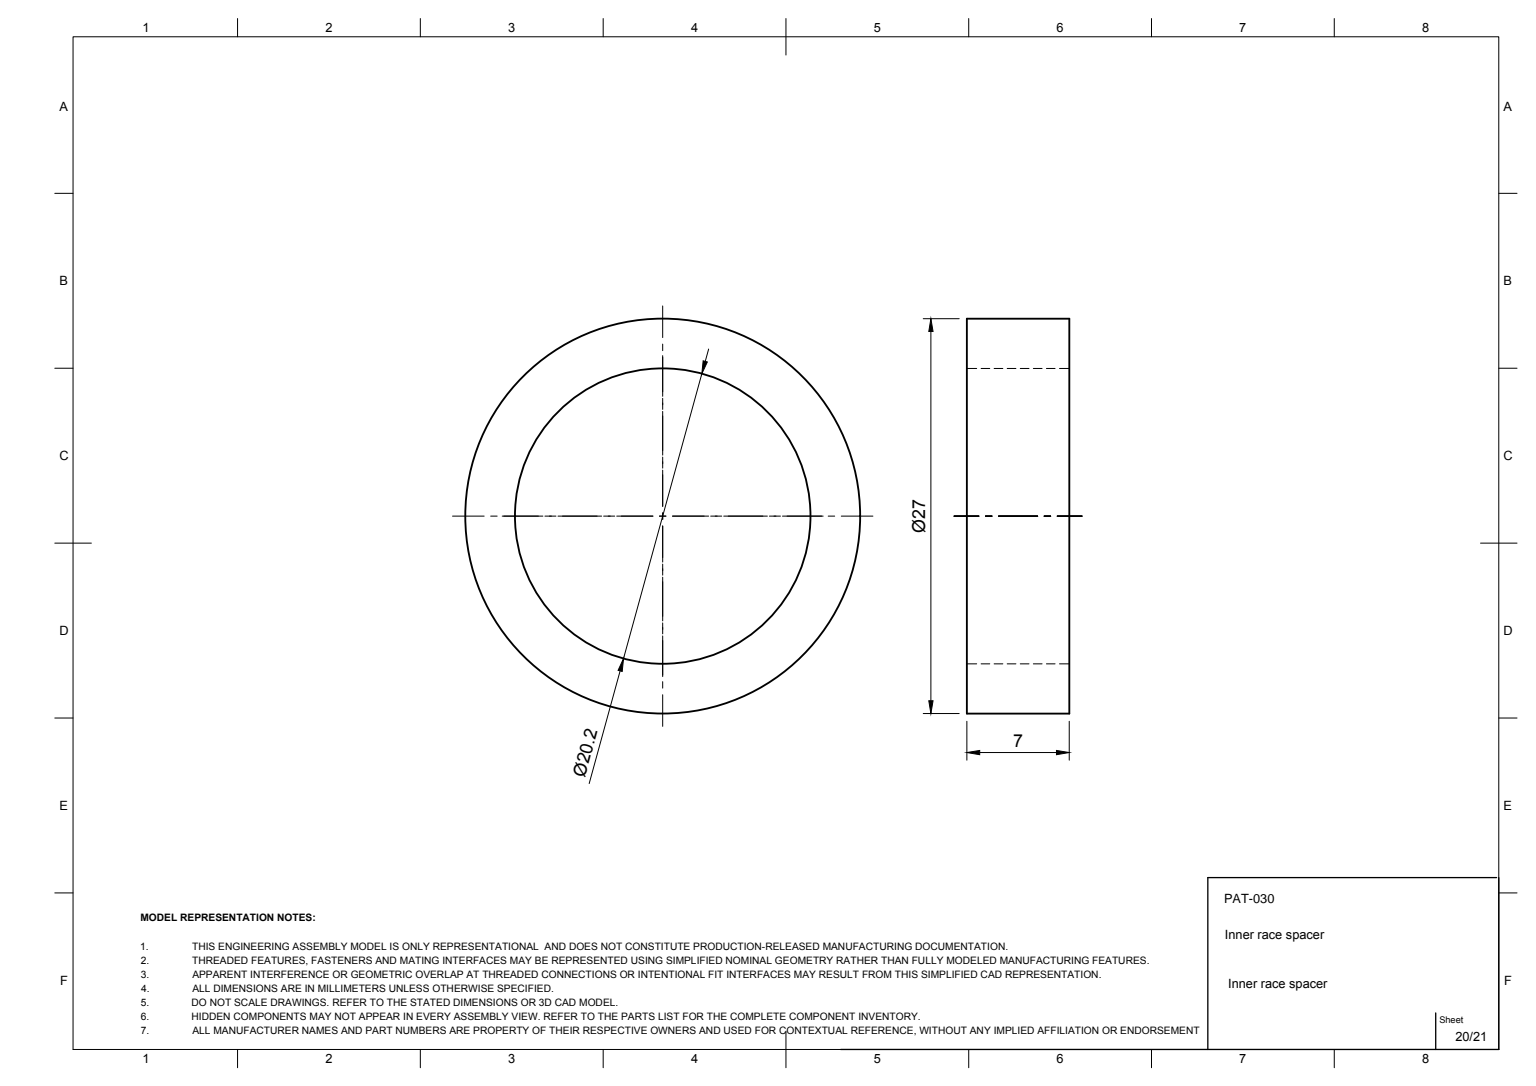
ISO-10303-21;
HEADER;
/* Generated by software containing ST-Developer
 * from STEP Tools, Inc. (www.steptools.com) 
 */

FILE_DESCRIPTION(
/* description */ ('Double-bearing flanged cartridge'),
/* implementation_level */ '2;1');

FILE_NAME(
/* name */ 'Inner race spacer.step',
/* time_stamp */ '2026-10-28T03:26:40-07:00',
/* author */ (''),
/* organization */ (''),
/* preprocessor_version */ 'ST-DEVELOPER v20.2',
/* originating_system */ 'Autodesk Translation Framework v15.17.0.0',
/* authorisation */ '');

FILE_SCHEMA (('AUTOMOTIVE_DESIGN { 1 0 10303 214 3 1 1 }'));
ENDSEC;

DATA;
#10=MECHANICAL_DESIGN_GEOMETRIC_PRESENTATION_REPRESENTATION('',(#210),#5535);
#174=SHAPE_REPRESENTATION_RELATIONSHIP('SRR','None',#5617,#188);
#188=ADVANCED_BREP_SHAPE_REPRESENTATION('',(#231),#5533);
#210=STYLED_ITEM('',(#5764),#231);
#231=MANIFOLD_SOLID_BREP('Body1',#2345);
#294=FACE_BOUND('',#711,.T.);
#295=FACE_BOUND('',#713,.T.);
#357=PLANE('',#2842);
#358=PLANE('',#2843);
#498=FACE_OUTER_BOUND('',#708,.T.);
#499=FACE_OUTER_BOUND('',#709,.T.);
#500=FACE_OUTER_BOUND('',#710,.T.);
#501=FACE_OUTER_BOUND('',#712,.T.);
#708=EDGE_LOOP('',(#2066,#2067,#2068,#2069));
#709=EDGE_LOOP('',(#2070,#2071,#2072,#2073));
#710=EDGE_LOOP('',(#2074));
#711=EDGE_LOOP('',(#2075));
#712=EDGE_LOOP('',(#2076));
#713=EDGE_LOOP('',(#2077));
#806=LINE('',#4637,#892);
#807=LINE('',#4643,#893);
#892=VECTOR('',#3619,1.01);
#893=VECTOR('',#3626,1.35);
#1058=CIRCLE('',#2837,1.01);
#1059=CIRCLE('',#2838,1.01);
#1060=CIRCLE('',#2840,1.35);
#1061=CIRCLE('',#2841,1.35);
#1252=VERTEX_POINT('',#4634);
#1253=VERTEX_POINT('',#4636);
#1254=VERTEX_POINT('',#4640);
#1255=VERTEX_POINT('',#4642);
#1526=EDGE_CURVE('',#1252,#1252,#1058,.T.);
#1527=EDGE_CURVE('',#1252,#1253,#806,.T.);
#1528=EDGE_CURVE('',#1253,#1253,#1059,.T.);
#1529=EDGE_CURVE('',#1254,#1254,#1060,.T.);
#1530=EDGE_CURVE('',#1254,#1255,#807,.T.);
#1531=EDGE_CURVE('',#1255,#1255,#1061,.T.);
#2066=ORIENTED_EDGE('',*,*,#1526,.F.);
#2067=ORIENTED_EDGE('',*,*,#1527,.T.);
#2068=ORIENTED_EDGE('',*,*,#1528,.T.);
#2069=ORIENTED_EDGE('',*,*,#1527,.F.);
#2070=ORIENTED_EDGE('',*,*,#1529,.F.);
#2071=ORIENTED_EDGE('',*,*,#1530,.T.);
#2072=ORIENTED_EDGE('',*,*,#1531,.T.);
#2073=ORIENTED_EDGE('',*,*,#1530,.F.);
#2074=ORIENTED_EDGE('',*,*,#1529,.T.);
#2075=ORIENTED_EDGE('',*,*,#1526,.T.);
#2076=ORIENTED_EDGE('',*,*,#1531,.F.);
#2077=ORIENTED_EDGE('',*,*,#1528,.F.);
#2168=CYLINDRICAL_SURFACE('',#2836,1.01);
#2169=CYLINDRICAL_SURFACE('',#2839,1.35);
#2312=ADVANCED_FACE('',(#498),#2168,.F.);
#2313=ADVANCED_FACE('',(#499),#2169,.T.);
#2314=ADVANCED_FACE('',(#500,#294),#357,.T.);
#2315=ADVANCED_FACE('',(#501,#295),#358,.F.);
#2345=CLOSED_SHELL('',(#2312,#2313,#2314,#2315));
#2835=AXIS2_PLACEMENT_3D('',#4632,#3613,#3614);
#2836=AXIS2_PLACEMENT_3D('',#4633,#3615,#3616);
#2837=AXIS2_PLACEMENT_3D('',#4635,#3617,#3618);
#2838=AXIS2_PLACEMENT_3D('',#4638,#3620,#3621);
#2839=AXIS2_PLACEMENT_3D('',#4639,#3622,#3623);
#2840=AXIS2_PLACEMENT_3D('',#4641,#3624,#3625);
#2841=AXIS2_PLACEMENT_3D('',#4644,#3627,#3628);
#2842=AXIS2_PLACEMENT_3D('',#4645,#3629,#3630);
#2843=AXIS2_PLACEMENT_3D('',#4646,#3631,#3632);
#3613=DIRECTION('axis',(0.,0.,1.));
#3614=DIRECTION('refdir',(1.,0.,0.));
#3615=DIRECTION('center_axis',(0.,1.,0.));
#3616=DIRECTION('ref_axis',(1.,0.,0.));
#3617=DIRECTION('center_axis',(0.,-1.,0.));
#3618=DIRECTION('ref_axis',(1.,0.,0.));
#3619=DIRECTION('',(0.,-1.,0.));
#3620=DIRECTION('center_axis',(0.,-1.,0.));
#3621=DIRECTION('ref_axis',(1.,0.,0.));
#3622=DIRECTION('center_axis',(0.,1.,0.));
#3623=DIRECTION('ref_axis',(1.,0.,0.));
#3624=DIRECTION('center_axis',(0.,1.,0.));
#3625=DIRECTION('ref_axis',(1.,0.,0.));
#3626=DIRECTION('',(0.,-1.,0.));
#3627=DIRECTION('center_axis',(0.,1.,0.));
#3628=DIRECTION('ref_axis',(1.,0.,0.));
#3629=DIRECTION('center_axis',(0.,1.,0.));
#3630=DIRECTION('ref_axis',(1.,0.,0.));
#3631=DIRECTION('center_axis',(0.,1.,0.));
#3632=DIRECTION('ref_axis',(1.,0.,0.));
#4632=CARTESIAN_POINT('',(0.,0.,0.));
#4633=CARTESIAN_POINT('Origin',(0.,5.7,4.5));
#4634=CARTESIAN_POINT('',(-1.01,6.4,4.5));
#4635=CARTESIAN_POINT('Origin',(0.,6.4,4.5));
#4636=CARTESIAN_POINT('',(-1.01,5.7,4.5));
#4637=CARTESIAN_POINT('',(-1.01,5.7,4.5));
#4638=CARTESIAN_POINT('Origin',(0.,5.7,4.5));
#4639=CARTESIAN_POINT('Origin',(0.,5.7,4.5));
#4640=CARTESIAN_POINT('',(-1.35,6.4,4.5));
#4641=CARTESIAN_POINT('Origin',(0.,6.4,4.5));
#4642=CARTESIAN_POINT('',(-1.35,5.7,4.5));
#4643=CARTESIAN_POINT('',(-1.35,5.7,4.5));
#4644=CARTESIAN_POINT('Origin',(0.,5.7,4.5));
#4645=CARTESIAN_POINT('Origin',(0.,6.4,4.5));
#4646=CARTESIAN_POINT('Origin',(0.,5.7,4.5));
#5514=UNCERTAINTY_MEASURE_WITH_UNIT(LENGTH_MEASURE(0.001),#5536,
'DISTANCE_ACCURACY_VALUE',
'Maximum model space distance between geometric entities at asserted c
onnectivities');
#5516=UNCERTAINTY_MEASURE_WITH_UNIT(LENGTH_MEASURE(0.001),#5536,
'DISTANCE_ACCURACY_VALUE',
'Maximum model space distance between geometric entities at asserted c
onnectivities');
#5533=(
GEOMETRIC_REPRESENTATION_CONTEXT(3)
GLOBAL_UNCERTAINTY_ASSIGNED_CONTEXT((#5514))
GLOBAL_UNIT_ASSIGNED_CONTEXT((#5536,#5538,#5539))
REPRESENTATION_CONTEXT('','3D')
);
#5535=(
GEOMETRIC_REPRESENTATION_CONTEXT(3)
GLOBAL_UNCERTAINTY_ASSIGNED_CONTEXT((#5516))
GLOBAL_UNIT_ASSIGNED_CONTEXT((#5536,#5538,#5539))
REPRESENTATION_CONTEXT('','3D')
);
#5536=(
LENGTH_UNIT()
NAMED_UNIT(*)
SI_UNIT(.CENTI.,.METRE.)
);
#5538=(
NAMED_UNIT(*)
PLANE_ANGLE_UNIT()
SI_UNIT($,.RADIAN.)
);
#5539=(
NAMED_UNIT(*)
SI_UNIT($,.STERADIAN.)
SOLID_ANGLE_UNIT()
);
#5556=SHAPE_DEFINITION_REPRESENTATION(#5594,#5617);
#5594=PRODUCT_DEFINITION_SHAPE('',$,#5636);
#5617=SHAPE_REPRESENTATION('',(#2835),#5533);
#5619=PRODUCT_DEFINITION_CONTEXT('part definition',#5675,'design');
#5636=PRODUCT_DEFINITION('Inner race spacer','Inner race spacer',#5654,
#5619);
#5654=PRODUCT_DEFINITION_FORMATION('',$,#5693);
#5675=APPLICATION_CONTEXT(
'Core Data for Automotive Mechanical Design Process');
#5676=PRODUCT_CONTEXT('part definition',#5675,'mechanical');
#5693=PRODUCT('Inner race spacer','Inner race spacer',
'Inner race spacer',(#5676));
#5758=COLOUR_RGB('Grey',0.48,0.52,0.57);
#5759=FILL_AREA_STYLE_COLOUR('',#5758);
#5760=FILL_AREA_STYLE('',(#5759));
#5761=SURFACE_STYLE_FILL_AREA(#5760);
#5762=SURFACE_SIDE_STYLE('',(#5761));
#5763=SURFACE_STYLE_USAGE(.BOTH.,#5762);
#5764=PRESENTATION_STYLE_ASSIGNMENT((#5763));
ENDSEC;
END-ISO-10303-21;
